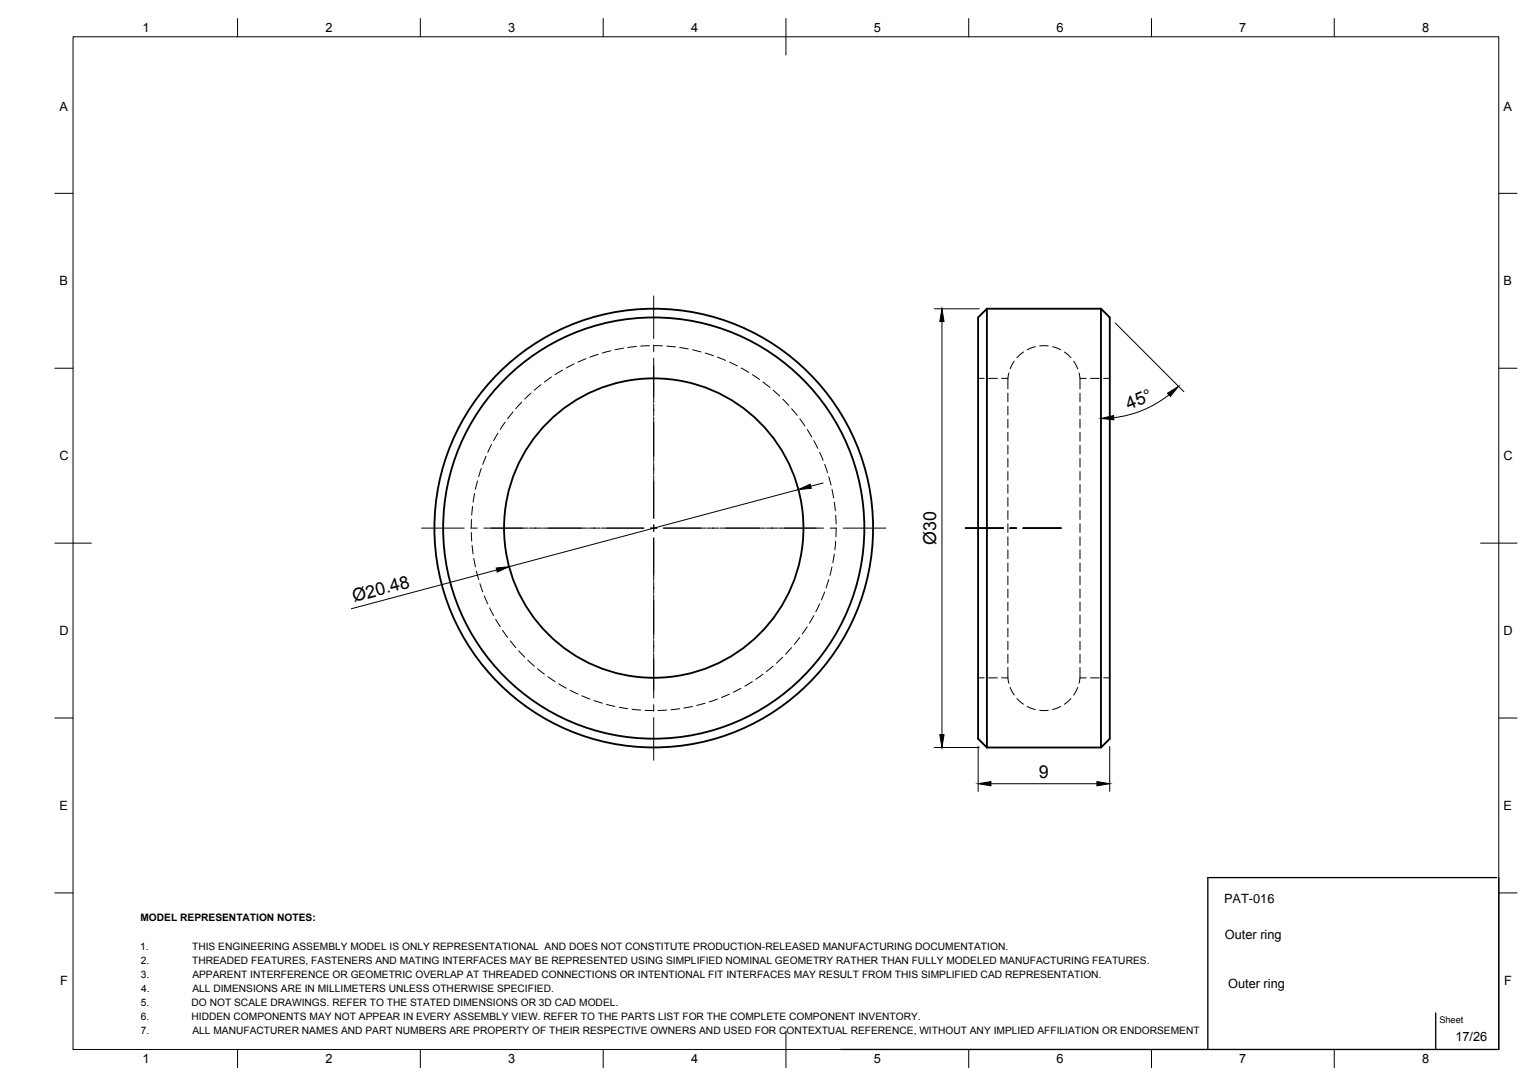
ISO-10303-21;
HEADER;
/* Generated by software containing ST-Developer
 * from STEP Tools, Inc. (www.steptools.com) 
 */

FILE_DESCRIPTION(
/* description */ ('Bracket-mounted idler roller'),
/* implementation_level */ '2;1');

FILE_NAME(
/* name */ 'Outer ring.step',
/* time_stamp */ '2026-10-28T03:26:42-07:00',
/* author */ (''),
/* organization */ (''),
/* preprocessor_version */ 'ST-DEVELOPER v20.2',
/* originating_system */ 'Autodesk Translation Framework v15.17.0.0',
/* authorisation */ '');

FILE_SCHEMA (('AUTOMOTIVE_DESIGN { 1 0 10303 214 3 1 1 }'));
ENDSEC;

DATA;
#10=MECHANICAL_DESIGN_GEOMETRIC_PRESENTATION_REPRESENTATION('',(#292),#6241);
#222=TOROIDAL_SURFACE('',#3628,1.,0.247676);
#228=CONICAL_SURFACE('',#3639,1.47,0.785398163397449);
#229=CONICAL_SURFACE('',#3643,1.47,0.785398163397449);
#250=SHAPE_REPRESENTATION_RELATIONSHIP('SRR','None',#6355,#271);
#271=ADVANCED_BREP_SHAPE_REPRESENTATION('',(#320),#6231);
#292=STYLED_ITEM('',(#6538),#320);
#320=MANIFOLD_SOLID_BREP('Body1',#3195);
#375=FACE_BOUND('',#848,.T.);
#376=FACE_BOUND('',#853,.T.);
#480=PLANE('',#3636);
#481=PLANE('',#3645);
#615=FACE_OUTER_BOUND('',#845,.T.);
#616=FACE_OUTER_BOUND('',#846,.T.);
#617=FACE_OUTER_BOUND('',#847,.T.);
#618=FACE_OUTER_BOUND('',#849,.T.);
#619=FACE_OUTER_BOUND('',#850,.T.);
#620=FACE_OUTER_BOUND('',#851,.T.);
#621=FACE_OUTER_BOUND('',#852,.T.);
#622=FACE_OUTER_BOUND('',#854,.T.);
#845=EDGE_LOOP('',(#2552,#2553,#2554,#2555,#2556,#2557));
#846=EDGE_LOOP('',(#2558,#2559,#2560,#2561,#2562));
#847=EDGE_LOOP('',(#2563));
#848=EDGE_LOOP('',(#2564));
#849=EDGE_LOOP('',(#2565,#2566,#2567,#2568));
#850=EDGE_LOOP('',(#2569,#2570,#2571,#2572));
#851=EDGE_LOOP('',(#2573,#2574,#2575,#2576));
#852=EDGE_LOOP('',(#2577));
#853=EDGE_LOOP('',(#2578));
#854=EDGE_LOOP('',(#2579,#2580,#2581,#2582,#2583));
#1104=LINE('',#5398,#1286);
#1105=LINE('',#5407,#1287);
#1106=LINE('',#5411,#1288);
#1107=LINE('',#5415,#1289);
#1108=LINE('',#5418,#1290);
#1286=VECTOR('',#4393,1.023815);
#1287=VECTOR('',#4404,1.47);
#1288=VECTOR('',#4409,1.5);
#1289=VECTOR('',#4414,1.47);
#1290=VECTOR('',#4419,1.023815);
#1411=CIRCLE('',#3629,1.023815);
#1412=CIRCLE('',#3630,1.023815);
#1413=CIRCLE('',#3631,0.247676);
#1414=CIRCLE('',#3632,1.023815);
#1415=CIRCLE('',#3633,1.023815);
#1416=CIRCLE('',#3635,1.023815);
#1417=CIRCLE('',#3637,1.44);
#1418=CIRCLE('',#3638,1.023815);
#1419=CIRCLE('',#3640,1.5);
#1420=CIRCLE('',#3642,1.5);
#1421=CIRCLE('',#3644,1.44);
#1651=VERTEX_POINT('',#5386);
#1652=VERTEX_POINT('',#5387);
#1653=VERTEX_POINT('',#5390);
#1654=VERTEX_POINT('',#5392);
#1655=VERTEX_POINT('',#5396);
#1656=VERTEX_POINT('',#5400);
#1657=VERTEX_POINT('',#5402);
#1658=VERTEX_POINT('',#5405);
#1659=VERTEX_POINT('',#5409);
#1660=VERTEX_POINT('',#5413);
#1978=EDGE_CURVE('',#1651,#1652,#1411,.T.);
#1979=EDGE_CURVE('',#1652,#1651,#1412,.T.);
#1980=EDGE_CURVE('',#1652,#1653,#1413,.T.);
#1981=EDGE_CURVE('',#1654,#1653,#1414,.T.);
#1982=EDGE_CURVE('',#1653,#1654,#1415,.T.);
#1983=EDGE_CURVE('',#1655,#1655,#1416,.T.);
#1984=EDGE_CURVE('',#1655,#1654,#1104,.T.);
#1985=EDGE_CURVE('',#1656,#1656,#1417,.T.);
#1986=EDGE_CURVE('',#1657,#1657,#1418,.T.);
#1987=EDGE_CURVE('',#1658,#1658,#1419,.T.);
#1988=EDGE_CURVE('',#1658,#1656,#1105,.T.);
#1989=EDGE_CURVE('',#1659,#1659,#1420,.T.);
#1990=EDGE_CURVE('',#1659,#1658,#1106,.T.);
#1991=EDGE_CURVE('',#1660,#1660,#1421,.T.);
#1992=EDGE_CURVE('',#1660,#1659,#1107,.T.);
#1993=EDGE_CURVE('',#1651,#1657,#1108,.T.);
#2552=ORIENTED_EDGE('',*,*,#1978,.F.);
#2553=ORIENTED_EDGE('',*,*,#1979,.F.);
#2554=ORIENTED_EDGE('',*,*,#1980,.T.);
#2555=ORIENTED_EDGE('',*,*,#1981,.F.);
#2556=ORIENTED_EDGE('',*,*,#1982,.F.);
#2557=ORIENTED_EDGE('',*,*,#1980,.F.);
#2558=ORIENTED_EDGE('',*,*,#1983,.T.);
#2559=ORIENTED_EDGE('',*,*,#1984,.T.);
#2560=ORIENTED_EDGE('',*,*,#1981,.T.);
#2561=ORIENTED_EDGE('',*,*,#1982,.T.);
#2562=ORIENTED_EDGE('',*,*,#1984,.F.);
#2563=ORIENTED_EDGE('',*,*,#1985,.F.);
#2564=ORIENTED_EDGE('',*,*,#1986,.T.);
#2565=ORIENTED_EDGE('',*,*,#1987,.F.);
#2566=ORIENTED_EDGE('',*,*,#1988,.T.);
#2567=ORIENTED_EDGE('',*,*,#1985,.T.);
#2568=ORIENTED_EDGE('',*,*,#1988,.F.);
#2569=ORIENTED_EDGE('',*,*,#1989,.F.);
#2570=ORIENTED_EDGE('',*,*,#1990,.T.);
#2571=ORIENTED_EDGE('',*,*,#1987,.T.);
#2572=ORIENTED_EDGE('',*,*,#1990,.F.);
#2573=ORIENTED_EDGE('',*,*,#1991,.F.);
#2574=ORIENTED_EDGE('',*,*,#1992,.T.);
#2575=ORIENTED_EDGE('',*,*,#1989,.T.);
#2576=ORIENTED_EDGE('',*,*,#1992,.F.);
#2577=ORIENTED_EDGE('',*,*,#1991,.T.);
#2578=ORIENTED_EDGE('',*,*,#1983,.F.);
#2579=ORIENTED_EDGE('',*,*,#1978,.T.);
#2580=ORIENTED_EDGE('',*,*,#1979,.T.);
#2581=ORIENTED_EDGE('',*,*,#1993,.T.);
#2582=ORIENTED_EDGE('',*,*,#1986,.F.);
#2583=ORIENTED_EDGE('',*,*,#1993,.F.);
#2958=CYLINDRICAL_SURFACE('',#3634,1.023815);
#2959=CYLINDRICAL_SURFACE('',#3641,1.5);
#2960=CYLINDRICAL_SURFACE('',#3646,1.023815);
#3090=ADVANCED_FACE('',(#615),#222,.F.);
#3091=ADVANCED_FACE('',(#616),#2958,.F.);
#3092=ADVANCED_FACE('',(#617,#375),#480,.T.);
#3093=ADVANCED_FACE('',(#618),#228,.T.);
#3094=ADVANCED_FACE('',(#619),#2959,.T.);
#3095=ADVANCED_FACE('',(#620),#229,.T.);
#3096=ADVANCED_FACE('',(#621,#376),#481,.T.);
#3097=ADVANCED_FACE('',(#622),#2960,.F.);
#3195=CLOSED_SHELL('',(#3090,#3091,#3092,#3093,#3094,#3095,#3096,#3097));
#3627=AXIS2_PLACEMENT_3D('',#5384,#4375,#4376);
#3628=AXIS2_PLACEMENT_3D('',#5385,#4377,#4378);
#3629=AXIS2_PLACEMENT_3D('',#5388,#4379,#4380);
#3630=AXIS2_PLACEMENT_3D('',#5389,#4381,#4382);
#3631=AXIS2_PLACEMENT_3D('',#5391,#4383,#4384);
#3632=AXIS2_PLACEMENT_3D('',#5393,#4385,#4386);
#3633=AXIS2_PLACEMENT_3D('',#5394,#4387,#4388);
#3634=AXIS2_PLACEMENT_3D('',#5395,#4389,#4390);
#3635=AXIS2_PLACEMENT_3D('',#5397,#4391,#4392);
#3636=AXIS2_PLACEMENT_3D('',#5399,#4394,#4395);
#3637=AXIS2_PLACEMENT_3D('',#5401,#4396,#4397);
#3638=AXIS2_PLACEMENT_3D('',#5403,#4398,#4399);
#3639=AXIS2_PLACEMENT_3D('',#5404,#4400,#4401);
#3640=AXIS2_PLACEMENT_3D('',#5406,#4402,#4403);
#3641=AXIS2_PLACEMENT_3D('',#5408,#4405,#4406);
#3642=AXIS2_PLACEMENT_3D('',#5410,#4407,#4408);
#3643=AXIS2_PLACEMENT_3D('',#5412,#4410,#4411);
#3644=AXIS2_PLACEMENT_3D('',#5414,#4412,#4413);
#3645=AXIS2_PLACEMENT_3D('',#5416,#4415,#4416);
#3646=AXIS2_PLACEMENT_3D('',#5417,#4417,#4418);
#4375=DIRECTION('axis',(0.,0.,1.));
#4376=DIRECTION('refdir',(1.,0.,0.));
#4377=DIRECTION('center_axis',(0.,-1.,0.));
#4378=DIRECTION('ref_axis',(0.,0.,-1.));
#4379=DIRECTION('center_axis',(0.,-1.,0.));
#4380=DIRECTION('ref_axis',(1.,0.,0.));
#4381=DIRECTION('center_axis',(0.,-1.,0.));
#4382=DIRECTION('ref_axis',(1.,0.,0.));
#4383=DIRECTION('center_axis',(1.,0.,1.22464679914735E-16));
#4384=DIRECTION('ref_axis',(-1.22464679914735E-16,0.,1.));
#4385=DIRECTION('center_axis',(0.,1.,0.));
#4386=DIRECTION('ref_axis',(1.,0.,0.));
#4387=DIRECTION('center_axis',(0.,1.,0.));
#4388=DIRECTION('ref_axis',(1.,0.,0.));
#4389=DIRECTION('center_axis',(0.,-1.,0.));
#4390=DIRECTION('ref_axis',(1.,0.,0.));
#4391=DIRECTION('center_axis',(0.,-1.,0.));
#4392=DIRECTION('ref_axis',(1.,0.,0.));
#4393=DIRECTION('',(0.,1.,0.));
#4394=DIRECTION('center_axis',(0.,1.,0.));
#4395=DIRECTION('ref_axis',(0.,0.,1.));
#4396=DIRECTION('center_axis',(0.,-1.,0.));
#4397=DIRECTION('ref_axis',(1.,0.,0.));
#4398=DIRECTION('center_axis',(0.,-1.,0.));
#4399=DIRECTION('ref_axis',(1.,0.,0.));
#4400=DIRECTION('center_axis',(0.,-1.,0.));
#4401=DIRECTION('ref_axis',(1.,0.,0.));
#4402=DIRECTION('center_axis',(0.,-1.,0.));
#4403=DIRECTION('ref_axis',(1.,0.,0.));
#4404=DIRECTION('',(0.707106781186548,0.707106781186547,8.65956056235494E-17));
#4405=DIRECTION('center_axis',(0.,-1.,0.));
#4406=DIRECTION('ref_axis',(1.,0.,0.));
#4407=DIRECTION('center_axis',(0.,-1.,0.));
#4408=DIRECTION('ref_axis',(1.,0.,0.));
#4409=DIRECTION('',(0.,1.,0.));
#4410=DIRECTION('center_axis',(0.,1.,0.));
#4411=DIRECTION('ref_axis',(1.,0.,0.));
#4412=DIRECTION('center_axis',(0.,-1.,0.));
#4413=DIRECTION('ref_axis',(1.,0.,0.));
#4414=DIRECTION('',(-0.707106781186548,0.707106781186547,-8.65956056235494E-17));
#4415=DIRECTION('center_axis',(0.,-1.,0.));
#4416=DIRECTION('ref_axis',(0.,0.,-1.));
#4417=DIRECTION('center_axis',(0.,-1.,0.));
#4418=DIRECTION('ref_axis',(1.,0.,0.));
#4419=DIRECTION('',(0.,1.,0.));
#5384=CARTESIAN_POINT('',(0.,0.,0.));
#5385=CARTESIAN_POINT('Origin',(0.,0.,0.));
#5386=CARTESIAN_POINT('',(-1.023815,0.246528389340863,-1.25381176266905E-16));
#5387=CARTESIAN_POINT('',(-1.25381176266905E-16,0.246528389340863,1.023815));
#5388=CARTESIAN_POINT('Origin',(0.,0.246528389340863,0.));
#5389=CARTESIAN_POINT('Origin',(0.,0.246528389340863,0.));
#5390=CARTESIAN_POINT('',(-1.25381176266905E-16,-0.246528389340863,1.023815));
#5391=CARTESIAN_POINT('Origin',(-1.22464679914735E-16,0.,1.));
#5392=CARTESIAN_POINT('',(-1.023815,-0.246528389340863,1.25381176266905E-16));
#5393=CARTESIAN_POINT('Origin',(0.,-0.246528389340863,0.));
#5394=CARTESIAN_POINT('Origin',(0.,-0.246528389340863,0.));
#5395=CARTESIAN_POINT('Origin',(0.,0.,0.));
#5396=CARTESIAN_POINT('',(-1.023815,-0.45,-1.25381176266905E-16));
#5397=CARTESIAN_POINT('Origin',(0.,-0.45,0.));
#5398=CARTESIAN_POINT('',(-1.023815,0.,-1.25381176266905E-16));
#5399=CARTESIAN_POINT('Origin',(1.44,0.45,0.));
#5400=CARTESIAN_POINT('',(-1.44,0.45,-1.76349139077219E-16));
#5401=CARTESIAN_POINT('Origin',(0.,0.45,0.));
#5402=CARTESIAN_POINT('',(-1.023815,0.45,-1.25381176266905E-16));
#5403=CARTESIAN_POINT('Origin',(0.,0.45,0.));
#5404=CARTESIAN_POINT('Origin',(0.,0.42,0.));
#5405=CARTESIAN_POINT('',(-1.5,0.39,-1.83697019872103E-16));
#5406=CARTESIAN_POINT('Origin',(0.,0.39,0.));
#5407=CARTESIAN_POINT('',(-1.47,0.42,-1.80023079474661E-16));
#5408=CARTESIAN_POINT('Origin',(0.,0.,0.));
#5409=CARTESIAN_POINT('',(-1.5,-0.39,-1.83697019872103E-16));
#5410=CARTESIAN_POINT('Origin',(0.,-0.39,0.));
#5411=CARTESIAN_POINT('',(-1.5,0.,-1.83697019872103E-16));
#5412=CARTESIAN_POINT('Origin',(0.,-0.42,0.));
#5413=CARTESIAN_POINT('',(-1.44,-0.45,-1.76349139077219E-16));
#5414=CARTESIAN_POINT('Origin',(0.,-0.45,0.));
#5415=CARTESIAN_POINT('',(-1.47,-0.42,-1.80023079474661E-16));
#5416=CARTESIAN_POINT('Origin',(1.023815,-0.45,0.));
#5417=CARTESIAN_POINT('Origin',(0.,0.,0.));
#5418=CARTESIAN_POINT('',(-1.023815,0.,-1.25381176266905E-16));
#6205=UNCERTAINTY_MEASURE_WITH_UNIT(LENGTH_MEASURE(0.001),#6242,
'DISTANCE_ACCURACY_VALUE',
'Maximum model space distance between geometric entities at asserted c
onnectivities');
#6215=UNCERTAINTY_MEASURE_WITH_UNIT(LENGTH_MEASURE(0.001),#6242,
'DISTANCE_ACCURACY_VALUE',
'Maximum model space distance between geometric entities at asserted c
onnectivities');
#6231=(
GEOMETRIC_REPRESENTATION_CONTEXT(3)
GLOBAL_UNCERTAINTY_ASSIGNED_CONTEXT((#6205))
GLOBAL_UNIT_ASSIGNED_CONTEXT((#6242,#6244,#6245))
REPRESENTATION_CONTEXT('','3D')
);
#6241=(
GEOMETRIC_REPRESENTATION_CONTEXT(3)
GLOBAL_UNCERTAINTY_ASSIGNED_CONTEXT((#6215))
GLOBAL_UNIT_ASSIGNED_CONTEXT((#6242,#6244,#6245))
REPRESENTATION_CONTEXT('','3D')
);
#6242=(
LENGTH_UNIT()
NAMED_UNIT(*)
SI_UNIT(.CENTI.,.METRE.)
);
#6244=(
NAMED_UNIT(*)
PLANE_ANGLE_UNIT()
SI_UNIT($,.RADIAN.)
);
#6245=(
NAMED_UNIT(*)
SI_UNIT($,.STERADIAN.)
SOLID_ANGLE_UNIT()
);
#6261=SHAPE_DEFINITION_REPRESENTATION(#6286,#6355);
#6286=PRODUCT_DEFINITION_SHAPE('',$,#6381);
#6355=SHAPE_REPRESENTATION('',(#3627),#6231);
#6365=PRODUCT_DEFINITION_CONTEXT('part definition',#6442,'design');
#6381=PRODUCT_DEFINITION('Outer ring','Outer ring',#6406,#6365);
#6406=PRODUCT_DEFINITION_FORMATION('',$,#6459);
#6442=APPLICATION_CONTEXT(
'Core Data for Automotive Mechanical Design Process');
#6443=PRODUCT_CONTEXT('part definition',#6442,'mechanical');
#6459=PRODUCT('Outer ring','Outer ring','Outer ring',(#6443));
#6532=COLOUR_RGB('Grey',0.48,0.52,0.57);
#6533=FILL_AREA_STYLE_COLOUR('',#6532);
#6534=FILL_AREA_STYLE('',(#6533));
#6535=SURFACE_STYLE_FILL_AREA(#6534);
#6536=SURFACE_SIDE_STYLE('',(#6535));
#6537=SURFACE_STYLE_USAGE(.BOTH.,#6536);
#6538=PRESENTATION_STYLE_ASSIGNMENT((#6537));
ENDSEC;
END-ISO-10303-21;
